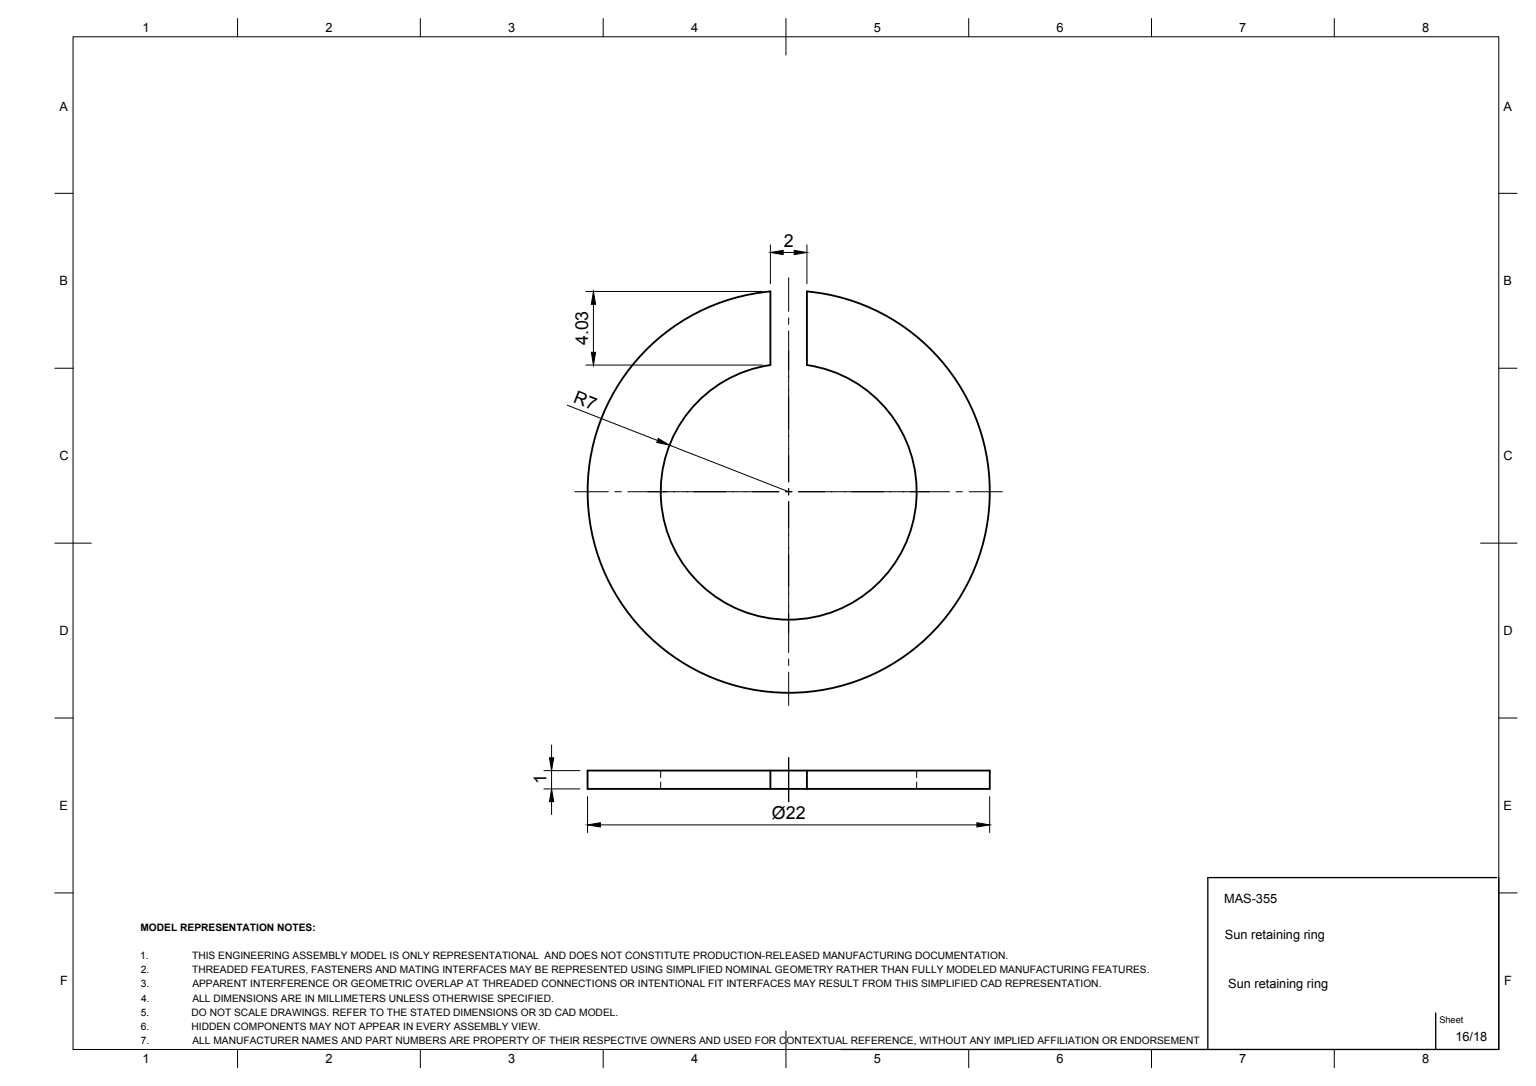
ISO-10303-21;
HEADER;
/* Generated by software containing ST-Developer
 * from STEP Tools, Inc. (www.steptools.com) 
 */

FILE_DESCRIPTION(
/* description */ ('Independent two-stage fixed-ring planetary gearbox,24/24/72 teeth,mod
ule2,20deg involutes,three planets per stage,4:1 x4:1=16:1. Native cut
-space/fillet/pattern tooth profiles derived from reusable gear blanks
; shared sun/planet/ring/carrier parts across both stages. Captured br
onze-journal input/carriers, headed retained planet pins, keyed inters
tage drive and modular keyed output interface. Native ideal gear links
; no torque, precision grade, production backlash/fits, lubrication, s
peed or life rating.'),
/* implementation_level */ '2;1');

FILE_NAME(
/* name */ 'Sun retaining ring.step',
/* time_stamp */ '2026-11-08T19:10:00-08:00',
/* author */ (''),
/* organization */ (''),
/* preprocessor_version */ 'ST-DEVELOPER v20.2',
/* originating_system */ 'Autodesk Translation Framework v15.17.0.0',
/* authorisation */ '');

FILE_SCHEMA (('AUTOMOTIVE_DESIGN { 1 0 10303 214 3 1 1 }'));
ENDSEC;

DATA;
#10=MECHANICAL_DESIGN_GEOMETRIC_PRESENTATION_REPRESENTATION('',(#1179),#259224);
#1139=SHAPE_REPRESENTATION_RELATIONSHIP('SRR','None',#259386,#1159);
#1159=ADVANCED_BREP_SHAPE_REPRESENTATION('',(#1199),#259220);
#1179=STYLED_ITEM('',(#259489),#1199);
#1199=MANIFOLD_SOLID_BREP('Body1',#25166);
#1678=PLANE('',#27149);
#1679=PLANE('',#27150);
#1680=PLANE('',#27151);
#1681=PLANE('',#27158);
#2974=FACE_OUTER_BOUND('',#4433,.T.);
#2975=FACE_OUTER_BOUND('',#4434,.T.);
#2976=FACE_OUTER_BOUND('',#4435,.T.);
#2977=FACE_OUTER_BOUND('',#4436,.T.);
#2978=FACE_OUTER_BOUND('',#4437,.T.);
#2979=FACE_OUTER_BOUND('',#4438,.T.);
#4433=EDGE_LOOP('',(#22718,#22719,#22720,#22721));
#4434=EDGE_LOOP('',(#22722,#22723,#22724,#22725));
#4435=EDGE_LOOP('',(#22726,#22727,#22728,#22729));
#4436=EDGE_LOOP('',(#22730,#22731,#22732,#22733));
#4437=EDGE_LOOP('',(#22734,#22735,#22736,#22737));
#4438=EDGE_LOOP('',(#22738,#22739,#22740,#22741));
#5369=CIRCLE('',#27152,11.);
#5370=CIRCLE('',#27153,7.);
#5371=CIRCLE('',#27155,7.);
#5372=CIRCLE('',#27157,11.);
#7776=LINE('',#256049,#8961);
#7777=LINE('',#256051,#8962);
#7778=LINE('',#256053,#8963);
#7779=LINE('',#256054,#8964);
#7780=LINE('',#256058,#8965);
#7781=LINE('',#256060,#8966);
#7782=LINE('',#256062,#8967);
#7783=LINE('',#256063,#8968);
#8961=VECTOR('',#31961,10.);
#8962=VECTOR('',#31962,10.);
#8963=VECTOR('',#31963,10.);
#8964=VECTOR('',#31964,10.);
#8965=VECTOR('',#31967,10.);
#8966=VECTOR('',#31968,10.);
#8967=VECTOR('',#31969,10.);
#8968=VECTOR('',#31970,10.);
#11477=VERTEX_POINT('',#256047);
#11478=VERTEX_POINT('',#256048);
#11479=VERTEX_POINT('',#256050);
#11480=VERTEX_POINT('',#256052);
#11481=VERTEX_POINT('',#256056);
#11482=VERTEX_POINT('',#256057);
#11483=VERTEX_POINT('',#256059);
#11484=VERTEX_POINT('',#256061);
#15244=EDGE_CURVE('',#11477,#11478,#7776,.T.);
#15245=EDGE_CURVE('',#11479,#11477,#7777,.T.);
#15246=EDGE_CURVE('',#11480,#11479,#7778,.T.);
#15247=EDGE_CURVE('',#11478,#11480,#7779,.T.);
#15248=EDGE_CURVE('',#11481,#11482,#7780,.T.);
#15249=EDGE_CURVE('',#11483,#11481,#7781,.T.);
#15250=EDGE_CURVE('',#11484,#11483,#7782,.T.);
#15251=EDGE_CURVE('',#11482,#11484,#7783,.T.);
#15252=EDGE_CURVE('',#11479,#11484,#5369,.T.);
#15253=EDGE_CURVE('',#11482,#11477,#5370,.T.);
#15254=EDGE_CURVE('',#11481,#11478,#5371,.T.);
#15255=EDGE_CURVE('',#11480,#11483,#5372,.T.);
#22718=ORIENTED_EDGE('',*,*,#15244,.F.);
#22719=ORIENTED_EDGE('',*,*,#15245,.F.);
#22720=ORIENTED_EDGE('',*,*,#15246,.F.);
#22721=ORIENTED_EDGE('',*,*,#15247,.F.);
#22722=ORIENTED_EDGE('',*,*,#15248,.F.);
#22723=ORIENTED_EDGE('',*,*,#15249,.F.);
#22724=ORIENTED_EDGE('',*,*,#15250,.F.);
#22725=ORIENTED_EDGE('',*,*,#15251,.F.);
#22726=ORIENTED_EDGE('',*,*,#15251,.T.);
#22727=ORIENTED_EDGE('',*,*,#15252,.F.);
#22728=ORIENTED_EDGE('',*,*,#15245,.T.);
#22729=ORIENTED_EDGE('',*,*,#15253,.F.);
#22730=ORIENTED_EDGE('',*,*,#15248,.T.);
#22731=ORIENTED_EDGE('',*,*,#15253,.T.);
#22732=ORIENTED_EDGE('',*,*,#15244,.T.);
#22733=ORIENTED_EDGE('',*,*,#15254,.F.);
#22734=ORIENTED_EDGE('',*,*,#15250,.T.);
#22735=ORIENTED_EDGE('',*,*,#15255,.F.);
#22736=ORIENTED_EDGE('',*,*,#15246,.T.);
#22737=ORIENTED_EDGE('',*,*,#15252,.T.);
#22738=ORIENTED_EDGE('',*,*,#15249,.T.);
#22739=ORIENTED_EDGE('',*,*,#15254,.T.);
#22740=ORIENTED_EDGE('',*,*,#15247,.T.);
#22741=ORIENTED_EDGE('',*,*,#15255,.T.);
#23756=CYLINDRICAL_SURFACE('',#27154,7.);
#23757=CYLINDRICAL_SURFACE('',#27156,11.);
#25080=ADVANCED_FACE('',(#2974),#1678,.F.);
#25081=ADVANCED_FACE('',(#2975),#1679,.F.);
#25082=ADVANCED_FACE('',(#2976),#1680,.F.);
#25083=ADVANCED_FACE('',(#2977),#23756,.F.);
#25084=ADVANCED_FACE('',(#2978),#23757,.T.);
#25085=ADVANCED_FACE('',(#2979),#1681,.T.);
#25166=CLOSED_SHELL('',(#25080,#25081,#25082,#25083,#25084,#25085));
#27148=AXIS2_PLACEMENT_3D('',#256045,#31957,#31958);
#27149=AXIS2_PLACEMENT_3D('',#256046,#31959,#31960);
#27150=AXIS2_PLACEMENT_3D('',#256055,#31965,#31966);
#27151=AXIS2_PLACEMENT_3D('',#256064,#31971,#31972);
#27152=AXIS2_PLACEMENT_3D('',#256065,#31973,#31974);
#27153=AXIS2_PLACEMENT_3D('',#256066,#31975,#31976);
#27154=AXIS2_PLACEMENT_3D('',#256067,#31977,#31978);
#27155=AXIS2_PLACEMENT_3D('',#256068,#31979,#31980);
#27156=AXIS2_PLACEMENT_3D('',#256069,#31981,#31982);
#27157=AXIS2_PLACEMENT_3D('',#256070,#31983,#31984);
#27158=AXIS2_PLACEMENT_3D('',#256071,#31985,#31986);
#31957=DIRECTION('axis',(0.,0.,1.));
#31958=DIRECTION('refdir',(1.,0.,0.));
#31959=DIRECTION('center_axis',(-1.,0.,0.));
#31960=DIRECTION('ref_axis',(0.,1.,0.));
#31961=DIRECTION('',(0.,0.,1.));
#31962=DIRECTION('',(0.,-1.,0.));
#31963=DIRECTION('',(0.,0.,-1.));
#31964=DIRECTION('',(0.,1.,0.));
#31965=DIRECTION('center_axis',(1.,0.,0.));
#31966=DIRECTION('ref_axis',(0.,-1.,0.));
#31967=DIRECTION('',(0.,0.,-1.));
#31968=DIRECTION('',(0.,-1.,0.));
#31969=DIRECTION('',(0.,0.,1.));
#31970=DIRECTION('',(0.,1.,0.));
#31971=DIRECTION('center_axis',(0.,0.,1.));
#31972=DIRECTION('ref_axis',(1.,0.,0.));
#31973=DIRECTION('center_axis',(0.,0.,1.));
#31974=DIRECTION('ref_axis',(1.,0.,0.));
#31975=DIRECTION('center_axis',(0.,0.,-1.));
#31976=DIRECTION('ref_axis',(1.,0.,0.));
#31977=DIRECTION('center_axis',(0.,0.,1.));
#31978=DIRECTION('ref_axis',(6.12323399573677E-17,-1.,0.));
#31979=DIRECTION('center_axis',(0.,0.,-1.));
#31980=DIRECTION('ref_axis',(1.,0.,0.));
#31981=DIRECTION('center_axis',(0.,0.,1.));
#31982=DIRECTION('ref_axis',(6.12323399573677E-17,-1.,0.));
#31983=DIRECTION('center_axis',(0.,0.,1.));
#31984=DIRECTION('ref_axis',(1.,0.,0.));
#31985=DIRECTION('center_axis',(0.,0.,1.));
#31986=DIRECTION('ref_axis',(1.,0.,0.));
#256045=CARTESIAN_POINT('',(0.,0.,0.));
#256046=CARTESIAN_POINT('Origin',(-1.,0.,1.));
#256047=CARTESIAN_POINT('',(-1.,6.92820323027551,0.));
#256048=CARTESIAN_POINT('',(-1.,6.92820323027551,1.));
#256049=CARTESIAN_POINT('',(-1.,6.92820323027551,0.));
#256050=CARTESIAN_POINT('',(-1.,10.9544511501033,0.));
#256051=CARTESIAN_POINT('',(-1.,0.,0.));
#256052=CARTESIAN_POINT('',(-1.,10.9544511501033,1.));
#256053=CARTESIAN_POINT('',(-1.,10.9544511501033,0.));
#256054=CARTESIAN_POINT('',(-1.,0.,1.));
#256055=CARTESIAN_POINT('Origin',(1.,22.,1.));
#256056=CARTESIAN_POINT('',(1.,6.92820323027551,1.));
#256057=CARTESIAN_POINT('',(1.,6.92820323027551,0.));
#256058=CARTESIAN_POINT('',(1.,6.92820323027551,0.));
#256059=CARTESIAN_POINT('',(1.,10.9544511501033,1.));
#256060=CARTESIAN_POINT('',(1.,11.,1.));
#256061=CARTESIAN_POINT('',(1.,10.9544511501033,0.));
#256062=CARTESIAN_POINT('',(1.,10.9544511501033,0.));
#256063=CARTESIAN_POINT('',(1.,11.,0.));
#256064=CARTESIAN_POINT('Origin',(0.,0.,0.));
#256065=CARTESIAN_POINT('Origin',(0.,0.,0.));
#256066=CARTESIAN_POINT('Origin',(0.,0.,0.));
#256067=CARTESIAN_POINT('Origin',(0.,0.,0.));
#256068=CARTESIAN_POINT('Origin',(0.,0.,1.));
#256069=CARTESIAN_POINT('Origin',(0.,0.,0.));
#256070=CARTESIAN_POINT('Origin',(0.,0.,1.));
#256071=CARTESIAN_POINT('Origin',(0.,0.,1.));
#259198=UNCERTAINTY_MEASURE_WITH_UNIT(LENGTH_MEASURE(0.01),#259225,
'DISTANCE_ACCURACY_VALUE',
'Maximum model space distance between geometric entities at asserted c
onnectivities');
#259202=UNCERTAINTY_MEASURE_WITH_UNIT(LENGTH_MEASURE(0.01),#259225,
'DISTANCE_ACCURACY_VALUE',
'Maximum model space distance between geometric entities at asserted c
onnectivities');
#259220=(
GEOMETRIC_REPRESENTATION_CONTEXT(3)
GLOBAL_UNCERTAINTY_ASSIGNED_CONTEXT((#259198))
GLOBAL_UNIT_ASSIGNED_CONTEXT((#259225,#259227,#259228))
REPRESENTATION_CONTEXT('','3D')
);
#259224=(
GEOMETRIC_REPRESENTATION_CONTEXT(3)
GLOBAL_UNCERTAINTY_ASSIGNED_CONTEXT((#259202))
GLOBAL_UNIT_ASSIGNED_CONTEXT((#259225,#259227,#259228))
REPRESENTATION_CONTEXT('','3D')
);
#259225=(
LENGTH_UNIT()
NAMED_UNIT(*)
SI_UNIT(.MILLI.,.METRE.)
);
#259227=(
NAMED_UNIT(*)
PLANE_ANGLE_UNIT()
SI_UNIT($,.RADIAN.)
);
#259228=(
NAMED_UNIT(*)
SI_UNIT($,.STERADIAN.)
SOLID_ANGLE_UNIT()
);
#259246=SHAPE_DEFINITION_REPRESENTATION(#259267,#259386);
#259267=PRODUCT_DEFINITION_SHAPE('',$,#259408);
#259386=SHAPE_REPRESENTATION('',(#27148),#259220);
#259390=PRODUCT_DEFINITION_CONTEXT('part definition',#259455,'design');
#259408=PRODUCT_DEFINITION('Sun retaining ring','Sun retaining ring',#259429,
#259390);
#259429=PRODUCT_DEFINITION_FORMATION('',$,#259474);
#259455=APPLICATION_CONTEXT(
'Core Data for Automotive Mechanical Design Process');
#259456=PRODUCT_CONTEXT('part definition',#259455,'mechanical');
#259474=PRODUCT('Sun retaining ring','Sun retaining ring',$,(#259456));
#259489=PRESENTATION_STYLE_ASSIGNMENT((#259504));
#259504=SURFACE_STYLE_USAGE(.BOTH.,#259519);
#259519=SURFACE_SIDE_STYLE('',(#259534));
#259534=SURFACE_STYLE_FILL_AREA(#259549);
#259549=FILL_AREA_STYLE('Dark gray',(#259564));
#259564=FILL_AREA_STYLE_COLOUR('Dark gray',#259579);
#259579=COLOUR_RGB('Dark gray',0.250980392156863,0.282352941176471,0.32156862745098);
ENDSEC;
END-ISO-10303-21;
